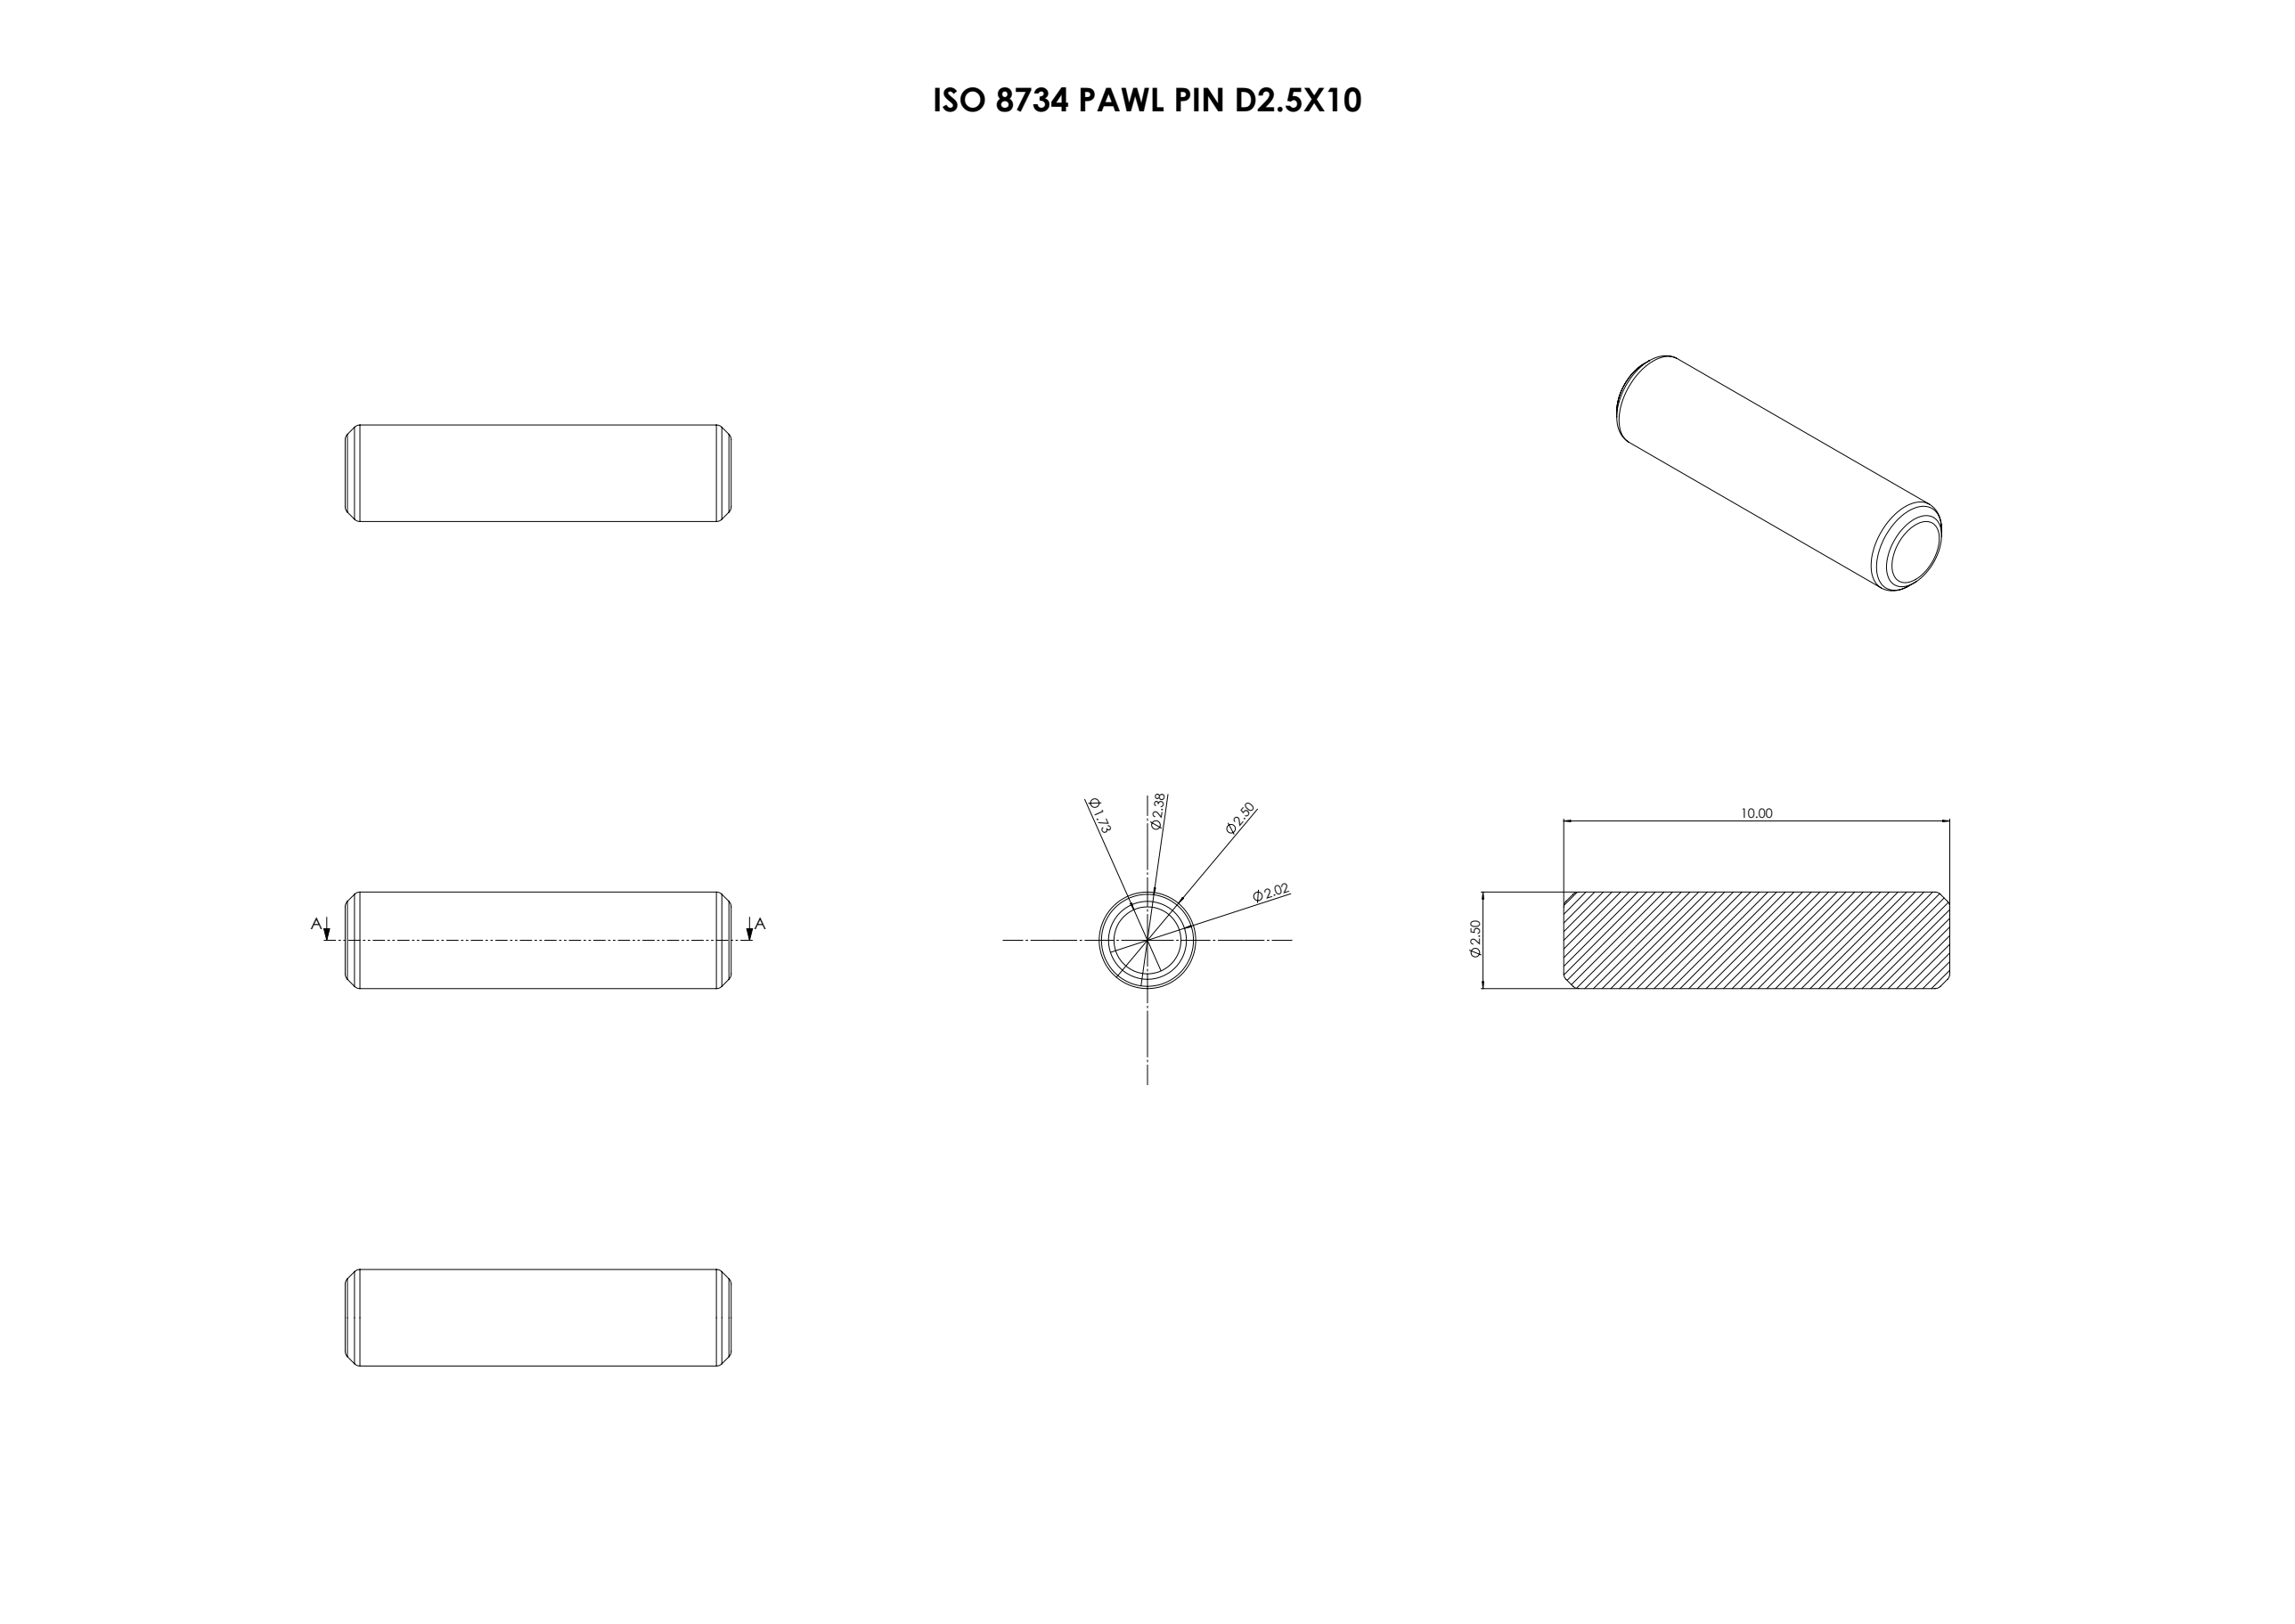
ISO-10303-21;
HEADER;
/* Generated by software containing ST-Developer
 * from STEP Tools, Inc. (www.steptools.com) 
 */

FILE_DESCRIPTION(
/* description */ (''),
/* implementation_level */ '2;1');

FILE_NAME(
/* name */ '06_ISO_8734_Pawl_Pin_D2.5x10.step',
/* time_stamp */ '2026-10-11T13:00:10-07:00',
/* author */ (''),
/* organization */ (''),
/* preprocessor_version */ 'ST-DEVELOPER v20.2',
/* originating_system */ 'Autodesk Translation Framework v15.15.0.0',
/* authorisation */ '');

FILE_SCHEMA (('AUTOMOTIVE_DESIGN { 1 0 10303 214 3 1 1 }'));
ENDSEC;

DATA;
#10=MECHANICAL_DESIGN_GEOMETRIC_PRESENTATION_REPRESENTATION('',(#363),#65563);
#155=TOROIDAL_SURFACE('',#21743,0.867157287525381,0.2);
#156=TOROIDAL_SURFACE('',#21752,1.05,0.2);
#157=TOROIDAL_SURFACE('',#21759,1.05,0.2);
#158=TOROIDAL_SURFACE('',#21766,0.867157287525381,0.2);
#341=SHAPE_REPRESENTATION_RELATIONSHIP('SRR','None',#65619,#352);
#352=ADVANCED_BREP_SHAPE_REPRESENTATION('',(#374),#65557);
#363=STYLED_ITEM('',(#65788),#374);
#374=MANIFOLD_SOLID_BREP('Body1',#20013);
#491=CONICAL_SURFACE('',#21748,1.1,0.785398163397448);
#492=CONICAL_SURFACE('',#21763,1.1,0.785398163397448);
#980=PLANE('',#21751);
#981=PLANE('',#21769);
#2004=FACE_OUTER_BOUND('',#3228,.T.);
#2005=FACE_OUTER_BOUND('',#3229,.T.);
#2006=FACE_OUTER_BOUND('',#3230,.T.);
#2007=FACE_OUTER_BOUND('',#3231,.T.);
#2008=FACE_OUTER_BOUND('',#3232,.T.);
#2009=FACE_OUTER_BOUND('',#3233,.T.);
#2010=FACE_OUTER_BOUND('',#3234,.T.);
#2011=FACE_OUTER_BOUND('',#3235,.T.);
#2012=FACE_OUTER_BOUND('',#3236,.T.);
#3228=EDGE_LOOP('',(#16816,#16817,#16818,#16819,#16820));
#3229=EDGE_LOOP('',(#16821,#16822,#16823,#16824,#16825,#16826));
#3230=EDGE_LOOP('',(#16827));
#3231=EDGE_LOOP('',(#16828,#16829,#16830,#16831,#16832,#16833));
#3232=EDGE_LOOP('',(#16834,#16835,#16836,#16837,#16838,#16839));
#3233=EDGE_LOOP('',(#16840,#16841,#16842,#16843,#16844,#16845));
#3234=EDGE_LOOP('',(#16846,#16847,#16848,#16849,#16850,#16851));
#3235=EDGE_LOOP('',(#16852,#16853,#16854,#16855,#16856));
#3236=EDGE_LOOP('',(#16857));
#4343=CIRCLE('',#21744,0.867157287525381);
#4344=CIRCLE('',#21745,0.2);
#4345=CIRCLE('',#21746,1.00857864376269);
#4346=CIRCLE('',#21747,1.00857864376269);
#4347=CIRCLE('',#21749,1.19142135623731);
#4348=CIRCLE('',#21750,1.19142135623731);
#4349=CIRCLE('',#21753,0.2);
#4350=CIRCLE('',#21754,1.25);
#4351=CIRCLE('',#21755,1.25);
#4352=CIRCLE('',#21757,1.25);
#4353=CIRCLE('',#21758,1.25);
#4354=CIRCLE('',#21760,0.2);
#4355=CIRCLE('',#21761,1.19142135623731);
#4356=CIRCLE('',#21762,1.19142135623731);
#4357=CIRCLE('',#21764,1.00857864376269);
#4358=CIRCLE('',#21765,1.00857864376269);
#4359=CIRCLE('',#21767,0.2);
#4360=CIRCLE('',#21768,0.867157287525381);
#6023=LINE('',#61957,#6915);
#6024=LINE('',#61970,#6916);
#6025=LINE('',#61982,#6917);
#6915=VECTOR('',#26200,1.1);
#6916=VECTOR('',#26217,1.25);
#6917=VECTOR('',#26232,1.1);
#8682=VERTEX_POINT('',#61948);
#8683=VERTEX_POINT('',#61950);
#8684=VERTEX_POINT('',#61952);
#8685=VERTEX_POINT('',#61956);
#8686=VERTEX_POINT('',#61958);
#8687=VERTEX_POINT('',#61963);
#8688=VERTEX_POINT('',#61965);
#8689=VERTEX_POINT('',#61969);
#8690=VERTEX_POINT('',#61971);
#8691=VERTEX_POINT('',#61975);
#8692=VERTEX_POINT('',#61977);
#8693=VERTEX_POINT('',#61981);
#8694=VERTEX_POINT('',#61983);
#8695=VERTEX_POINT('',#61987);
#11441=EDGE_CURVE('',#8682,#8682,#4343,.T.);
#11442=EDGE_CURVE('',#8682,#8683,#4344,.T.);
#11443=EDGE_CURVE('',#8683,#8684,#4345,.T.);
#11444=EDGE_CURVE('',#8684,#8683,#4346,.T.);
#11445=EDGE_CURVE('',#8684,#8685,#6023,.T.);
#11446=EDGE_CURVE('',#8686,#8685,#4347,.T.);
#11447=EDGE_CURVE('',#8685,#8686,#4348,.T.);
#11448=EDGE_CURVE('',#8686,#8687,#4349,.T.);
#11449=EDGE_CURVE('',#8687,#8688,#4350,.T.);
#11450=EDGE_CURVE('',#8688,#8687,#4351,.T.);
#11451=EDGE_CURVE('',#8688,#8689,#6024,.T.);
#11452=EDGE_CURVE('',#8690,#8689,#4352,.T.);
#11453=EDGE_CURVE('',#8689,#8690,#4353,.T.);
#11454=EDGE_CURVE('',#8690,#8691,#4354,.T.);
#11455=EDGE_CURVE('',#8691,#8692,#4355,.T.);
#11456=EDGE_CURVE('',#8692,#8691,#4356,.T.);
#11457=EDGE_CURVE('',#8692,#8693,#6025,.T.);
#11458=EDGE_CURVE('',#8694,#8693,#4357,.T.);
#11459=EDGE_CURVE('',#8693,#8694,#4358,.T.);
#11460=EDGE_CURVE('',#8694,#8695,#4359,.T.);
#11461=EDGE_CURVE('',#8695,#8695,#4360,.T.);
#16816=ORIENTED_EDGE('',*,*,#11441,.T.);
#16817=ORIENTED_EDGE('',*,*,#11442,.T.);
#16818=ORIENTED_EDGE('',*,*,#11443,.T.);
#16819=ORIENTED_EDGE('',*,*,#11444,.T.);
#16820=ORIENTED_EDGE('',*,*,#11442,.F.);
#16821=ORIENTED_EDGE('',*,*,#11444,.F.);
#16822=ORIENTED_EDGE('',*,*,#11445,.T.);
#16823=ORIENTED_EDGE('',*,*,#11446,.F.);
#16824=ORIENTED_EDGE('',*,*,#11447,.F.);
#16825=ORIENTED_EDGE('',*,*,#11445,.F.);
#16826=ORIENTED_EDGE('',*,*,#11443,.F.);
#16827=ORIENTED_EDGE('',*,*,#11441,.F.);
#16828=ORIENTED_EDGE('',*,*,#11446,.T.);
#16829=ORIENTED_EDGE('',*,*,#11447,.T.);
#16830=ORIENTED_EDGE('',*,*,#11448,.T.);
#16831=ORIENTED_EDGE('',*,*,#11449,.T.);
#16832=ORIENTED_EDGE('',*,*,#11450,.T.);
#16833=ORIENTED_EDGE('',*,*,#11448,.F.);
#16834=ORIENTED_EDGE('',*,*,#11450,.F.);
#16835=ORIENTED_EDGE('',*,*,#11451,.T.);
#16836=ORIENTED_EDGE('',*,*,#11452,.F.);
#16837=ORIENTED_EDGE('',*,*,#11453,.F.);
#16838=ORIENTED_EDGE('',*,*,#11451,.F.);
#16839=ORIENTED_EDGE('',*,*,#11449,.F.);
#16840=ORIENTED_EDGE('',*,*,#11452,.T.);
#16841=ORIENTED_EDGE('',*,*,#11453,.T.);
#16842=ORIENTED_EDGE('',*,*,#11454,.T.);
#16843=ORIENTED_EDGE('',*,*,#11455,.T.);
#16844=ORIENTED_EDGE('',*,*,#11456,.T.);
#16845=ORIENTED_EDGE('',*,*,#11454,.F.);
#16846=ORIENTED_EDGE('',*,*,#11456,.F.);
#16847=ORIENTED_EDGE('',*,*,#11457,.T.);
#16848=ORIENTED_EDGE('',*,*,#11458,.F.);
#16849=ORIENTED_EDGE('',*,*,#11459,.F.);
#16850=ORIENTED_EDGE('',*,*,#11457,.F.);
#16851=ORIENTED_EDGE('',*,*,#11455,.F.);
#16852=ORIENTED_EDGE('',*,*,#11458,.T.);
#16853=ORIENTED_EDGE('',*,*,#11459,.T.);
#16854=ORIENTED_EDGE('',*,*,#11460,.T.);
#16855=ORIENTED_EDGE('',*,*,#11461,.T.);
#16856=ORIENTED_EDGE('',*,*,#11460,.F.);
#16857=ORIENTED_EDGE('',*,*,#11461,.F.);
#18724=CYLINDRICAL_SURFACE('',#21756,1.25);
#19700=ADVANCED_FACE('',(#2004),#155,.T.);
#19701=ADVANCED_FACE('',(#2005),#491,.T.);
#19702=ADVANCED_FACE('',(#2006),#980,.T.);
#19703=ADVANCED_FACE('',(#2007),#156,.T.);
#19704=ADVANCED_FACE('',(#2008),#18724,.T.);
#19705=ADVANCED_FACE('',(#2009),#157,.T.);
#19706=ADVANCED_FACE('',(#2010),#492,.T.);
#19707=ADVANCED_FACE('',(#2011),#158,.T.);
#19708=ADVANCED_FACE('',(#2012),#981,.T.);
#20013=CLOSED_SHELL('',(#19700,#19701,#19702,#19703,#19704,#19705,#19706,
#19707,#19708));
#21742=AXIS2_PLACEMENT_3D('',#61946,#26186,#26187);
#21743=AXIS2_PLACEMENT_3D('',#61947,#26188,#26189);
#21744=AXIS2_PLACEMENT_3D('',#61949,#26190,#26191);
#21745=AXIS2_PLACEMENT_3D('',#61951,#26192,#26193);
#21746=AXIS2_PLACEMENT_3D('',#61953,#26194,#26195);
#21747=AXIS2_PLACEMENT_3D('',#61954,#26196,#26197);
#21748=AXIS2_PLACEMENT_3D('',#61955,#26198,#26199);
#21749=AXIS2_PLACEMENT_3D('',#61959,#26201,#26202);
#21750=AXIS2_PLACEMENT_3D('',#61960,#26203,#26204);
#21751=AXIS2_PLACEMENT_3D('',#61961,#26205,#26206);
#21752=AXIS2_PLACEMENT_3D('',#61962,#26207,#26208);
#21753=AXIS2_PLACEMENT_3D('',#61964,#26209,#26210);
#21754=AXIS2_PLACEMENT_3D('',#61966,#26211,#26212);
#21755=AXIS2_PLACEMENT_3D('',#61967,#26213,#26214);
#21756=AXIS2_PLACEMENT_3D('',#61968,#26215,#26216);
#21757=AXIS2_PLACEMENT_3D('',#61972,#26218,#26219);
#21758=AXIS2_PLACEMENT_3D('',#61973,#26220,#26221);
#21759=AXIS2_PLACEMENT_3D('',#61974,#26222,#26223);
#21760=AXIS2_PLACEMENT_3D('',#61976,#26224,#26225);
#21761=AXIS2_PLACEMENT_3D('',#61978,#26226,#26227);
#21762=AXIS2_PLACEMENT_3D('',#61979,#26228,#26229);
#21763=AXIS2_PLACEMENT_3D('',#61980,#26230,#26231);
#21764=AXIS2_PLACEMENT_3D('',#61984,#26233,#26234);
#21765=AXIS2_PLACEMENT_3D('',#61985,#26235,#26236);
#21766=AXIS2_PLACEMENT_3D('',#61986,#26237,#26238);
#21767=AXIS2_PLACEMENT_3D('',#61988,#26239,#26240);
#21768=AXIS2_PLACEMENT_3D('',#61989,#26241,#26242);
#21769=AXIS2_PLACEMENT_3D('',#61990,#26243,#26244);
#26186=DIRECTION('axis',(0.,0.,1.));
#26187=DIRECTION('refdir',(1.,0.,0.));
#26188=DIRECTION('center_axis',(1.,0.,0.));
#26189=DIRECTION('ref_axis',(0.,0.,-1.));
#26190=DIRECTION('center_axis',(-1.,0.,0.));
#26191=DIRECTION('ref_axis',(0.,-1.,1.83697019872103E-16));
#26192=DIRECTION('center_axis',(0.,-1.,-1.22464679914735E-16));
#26193=DIRECTION('ref_axis',(0.,-1.22464679914735E-16,1.));
#26194=DIRECTION('center_axis',(1.,0.,0.));
#26195=DIRECTION('ref_axis',(0.,-1.,3.06161699786838E-17));
#26196=DIRECTION('center_axis',(1.,0.,0.));
#26197=DIRECTION('ref_axis',(0.,-1.,3.06161699786838E-17));
#26198=DIRECTION('center_axis',(-1.,0.,0.));
#26199=DIRECTION('ref_axis',(0.,1.,0.));
#26200=DIRECTION('',(-0.707106781186548,-0.707106781186547,-8.65956056235493E-17));
#26201=DIRECTION('center_axis',(-1.,0.,0.));
#26202=DIRECTION('ref_axis',(0.,-1.,3.06161699786838E-17));
#26203=DIRECTION('center_axis',(-1.,0.,0.));
#26204=DIRECTION('ref_axis',(0.,-1.,3.06161699786838E-17));
#26205=DIRECTION('center_axis',(1.,0.,0.));
#26206=DIRECTION('ref_axis',(0.,0.,-1.));
#26207=DIRECTION('center_axis',(1.,0.,0.));
#26208=DIRECTION('ref_axis',(0.,0.,-1.));
#26209=DIRECTION('center_axis',(0.,-1.,-1.22464679914735E-16));
#26210=DIRECTION('ref_axis',(0.,-1.22464679914735E-16,1.));
#26211=DIRECTION('center_axis',(1.,0.,0.));
#26212=DIRECTION('ref_axis',(0.,-1.,1.83697019872103E-16));
#26213=DIRECTION('center_axis',(1.,0.,0.));
#26214=DIRECTION('ref_axis',(0.,-1.,1.83697019872103E-16));
#26215=DIRECTION('center_axis',(1.,0.,0.));
#26216=DIRECTION('ref_axis',(0.,1.,0.));
#26217=DIRECTION('',(-1.,0.,0.));
#26218=DIRECTION('center_axis',(-1.,0.,0.));
#26219=DIRECTION('ref_axis',(0.,-1.,1.83697019872103E-16));
#26220=DIRECTION('center_axis',(-1.,0.,0.));
#26221=DIRECTION('ref_axis',(0.,-1.,1.83697019872103E-16));
#26222=DIRECTION('center_axis',(1.,0.,0.));
#26223=DIRECTION('ref_axis',(0.,0.,-1.));
#26224=DIRECTION('center_axis',(0.,-1.,-1.22464679914735E-16));
#26225=DIRECTION('ref_axis',(0.,-1.22464679914735E-16,1.));
#26226=DIRECTION('center_axis',(1.,0.,0.));
#26227=DIRECTION('ref_axis',(0.,-1.,3.06161699786838E-17));
#26228=DIRECTION('center_axis',(1.,0.,0.));
#26229=DIRECTION('ref_axis',(0.,-1.,3.06161699786838E-17));
#26230=DIRECTION('center_axis',(1.,0.,0.));
#26231=DIRECTION('ref_axis',(0.,1.,0.));
#26232=DIRECTION('',(-0.707106781186547,0.707106781186547,8.65956056235493E-17));
#26233=DIRECTION('center_axis',(-1.,0.,0.));
#26234=DIRECTION('ref_axis',(0.,-1.,3.06161699786838E-17));
#26235=DIRECTION('center_axis',(-1.,0.,0.));
#26236=DIRECTION('ref_axis',(0.,-1.,3.06161699786838E-17));
#26237=DIRECTION('center_axis',(1.,0.,0.));
#26238=DIRECTION('ref_axis',(0.,0.,-1.));
#26239=DIRECTION('center_axis',(0.,-1.,-1.22464679914735E-16));
#26240=DIRECTION('ref_axis',(0.,-1.22464679914735E-16,1.));
#26241=DIRECTION('center_axis',(1.,0.,0.));
#26242=DIRECTION('ref_axis',(0.,-1.,1.83697019872103E-16));
#26243=DIRECTION('center_axis',(-1.,0.,0.));
#26244=DIRECTION('ref_axis',(0.,0.,1.));
#61946=CARTESIAN_POINT('',(0.,0.,0.));
#61947=CARTESIAN_POINT('Origin',(9.8,0.,0.));
#61948=CARTESIAN_POINT('',(10.,-1.06196139652526E-16,0.867157287525381));
#61949=CARTESIAN_POINT('Origin',(10.,0.,0.));
#61950=CARTESIAN_POINT('',(9.94142135623731,-1.23515260777236E-16,1.00857864376269));
#61951=CARTESIAN_POINT('Origin',(9.8,-1.06196139652526E-16,0.867157287525381));
#61952=CARTESIAN_POINT('',(9.94142135623731,-1.00857864376269,-1.23515260777236E-16));
#61953=CARTESIAN_POINT('Origin',(9.94142135623731,0.,-1.54394075971545E-16));
#61954=CARTESIAN_POINT('Origin',(9.94142135623731,0.,-1.54394075971545E-16));
#61955=CARTESIAN_POINT('Origin',(9.85,0.,0.));
#61956=CARTESIAN_POINT('',(9.75857864376269,-1.19142135623731,-1.45907035035182E-16));
#61957=CARTESIAN_POINT('',(9.85,-1.1,-1.34711147906209E-16));
#61958=CARTESIAN_POINT('',(9.75857864376269,-1.45907035035182E-16,1.19142135623731));
#61959=CARTESIAN_POINT('Origin',(9.75857864376269,0.,-1.82383793793977E-16));
#61960=CARTESIAN_POINT('Origin',(9.75857864376269,0.,-1.82383793793977E-16));
#61961=CARTESIAN_POINT('Origin',(10.,0.,0.));
#61962=CARTESIAN_POINT('Origin',(9.61715728752538,0.,0.));
#61963=CARTESIAN_POINT('',(9.61715728752538,-1.53080849893419E-16,1.25));
#61964=CARTESIAN_POINT('Origin',(9.61715728752538,-1.28587913910472E-16,
1.05));
#61965=CARTESIAN_POINT('',(9.61715728752538,-1.25,-1.53080849893419E-16));
#61966=CARTESIAN_POINT('Origin',(9.61715728752538,0.,0.));
#61967=CARTESIAN_POINT('Origin',(9.61715728752538,0.,0.));
#61968=CARTESIAN_POINT('Origin',(5.,0.,0.));
#61969=CARTESIAN_POINT('',(0.382842712474619,-1.25,-1.53080849893419E-16));
#61970=CARTESIAN_POINT('',(5.,-1.25,-1.53080849893419E-16));
#61971=CARTESIAN_POINT('',(0.382842712474619,-1.53080849893419E-16,1.25));
#61972=CARTESIAN_POINT('Origin',(0.382842712474619,0.,0.));
#61973=CARTESIAN_POINT('Origin',(0.382842712474619,0.,0.));
#61974=CARTESIAN_POINT('Origin',(0.382842712474619,0.,0.));
#61975=CARTESIAN_POINT('',(0.241421356237309,-1.45907035035182E-16,1.19142135623731));
#61976=CARTESIAN_POINT('Origin',(0.382842712474619,-1.28587913910472E-16,
1.05));
#61977=CARTESIAN_POINT('',(0.24142135623731,-1.19142135623731,-1.45907035035182E-16));
#61978=CARTESIAN_POINT('Origin',(0.241421356237309,0.,-1.82383793793977E-16));
#61979=CARTESIAN_POINT('Origin',(0.241421356237309,0.,-1.82383793793977E-16));
#61980=CARTESIAN_POINT('Origin',(0.15,0.,0.));
#61981=CARTESIAN_POINT('',(0.0585786437626904,-1.00857864376269,-1.23515260777236E-16));
#61982=CARTESIAN_POINT('',(0.15,-1.1,-1.34711147906209E-16));
#61983=CARTESIAN_POINT('',(0.0585786437626905,-1.23515260777236E-16,1.00857864376269));
#61984=CARTESIAN_POINT('Origin',(0.0585786437626905,0.,-1.54394075971545E-16));
#61985=CARTESIAN_POINT('Origin',(0.0585786437626905,0.,-1.54394075971545E-16));
#61986=CARTESIAN_POINT('Origin',(0.2,0.,0.));
#61987=CARTESIAN_POINT('',(0.,-1.06196139652526E-16,0.867157287525381));
#61988=CARTESIAN_POINT('Origin',(0.2,-1.06196139652526E-16,0.867157287525381));
#61989=CARTESIAN_POINT('Origin',(0.,0.,0.));
#61990=CARTESIAN_POINT('Origin',(0.,0.95,0.));
#65544=UNCERTAINTY_MEASURE_WITH_UNIT(LENGTH_MEASURE(0.01),#65564,
'DISTANCE_ACCURACY_VALUE',
'Maximum model space distance between geometric entities at asserted c
onnectivities');
#65550=UNCERTAINTY_MEASURE_WITH_UNIT(LENGTH_MEASURE(0.01),#65564,
'DISTANCE_ACCURACY_VALUE',
'Maximum model space distance between geometric entities at asserted c
onnectivities');
#65557=(
GEOMETRIC_REPRESENTATION_CONTEXT(3)
GLOBAL_UNCERTAINTY_ASSIGNED_CONTEXT((#65544))
GLOBAL_UNIT_ASSIGNED_CONTEXT((#65564,#65566,#65567))
REPRESENTATION_CONTEXT('','3D')
);
#65563=(
GEOMETRIC_REPRESENTATION_CONTEXT(3)
GLOBAL_UNCERTAINTY_ASSIGNED_CONTEXT((#65550))
GLOBAL_UNIT_ASSIGNED_CONTEXT((#65564,#65566,#65567))
REPRESENTATION_CONTEXT('','3D')
);
#65564=(
LENGTH_UNIT()
NAMED_UNIT(*)
SI_UNIT(.MILLI.,.METRE.)
);
#65566=(
NAMED_UNIT(*)
PLANE_ANGLE_UNIT()
SI_UNIT($,.RADIAN.)
);
#65567=(
NAMED_UNIT(*)
SI_UNIT($,.STERADIAN.)
SOLID_ANGLE_UNIT()
);
#65574=SHAPE_DEFINITION_REPRESENTATION(#65586,#65619);
#65586=PRODUCT_DEFINITION_SHAPE('',$,#65632);
#65619=SHAPE_REPRESENTATION('',(#21742),#65557);
#65625=PRODUCT_DEFINITION_CONTEXT('part definition',#65663,'design');
#65632=PRODUCT_DEFINITION('2026-10-10-05-45-28-330',
'06_ISO_8734_Pawl_Pin_D2.5x10',#65644,#65625);
#65644=PRODUCT_DEFINITION_FORMATION('',$,#65671);
#65663=APPLICATION_CONTEXT(
'Core Data for Automotive Mechanical Design Process');
#65664=PRODUCT_CONTEXT('part definition',#65663,'mechanical');
#65671=PRODUCT('2026-10-10-05-45-28-330','06_ISO_8734_Pawl_Pin_D2.5x10',
$,(#65664));
#65782=COLOUR_RGB('Grey',0.48,0.52,0.57);
#65783=FILL_AREA_STYLE_COLOUR('',#65782);
#65784=FILL_AREA_STYLE('',(#65783));
#65785=SURFACE_STYLE_FILL_AREA(#65784);
#65786=SURFACE_SIDE_STYLE('',(#65785));
#65787=SURFACE_STYLE_USAGE(.BOTH.,#65786);
#65788=PRESENTATION_STYLE_ASSIGNMENT((#65787));
ENDSEC;
END-ISO-10303-21;
